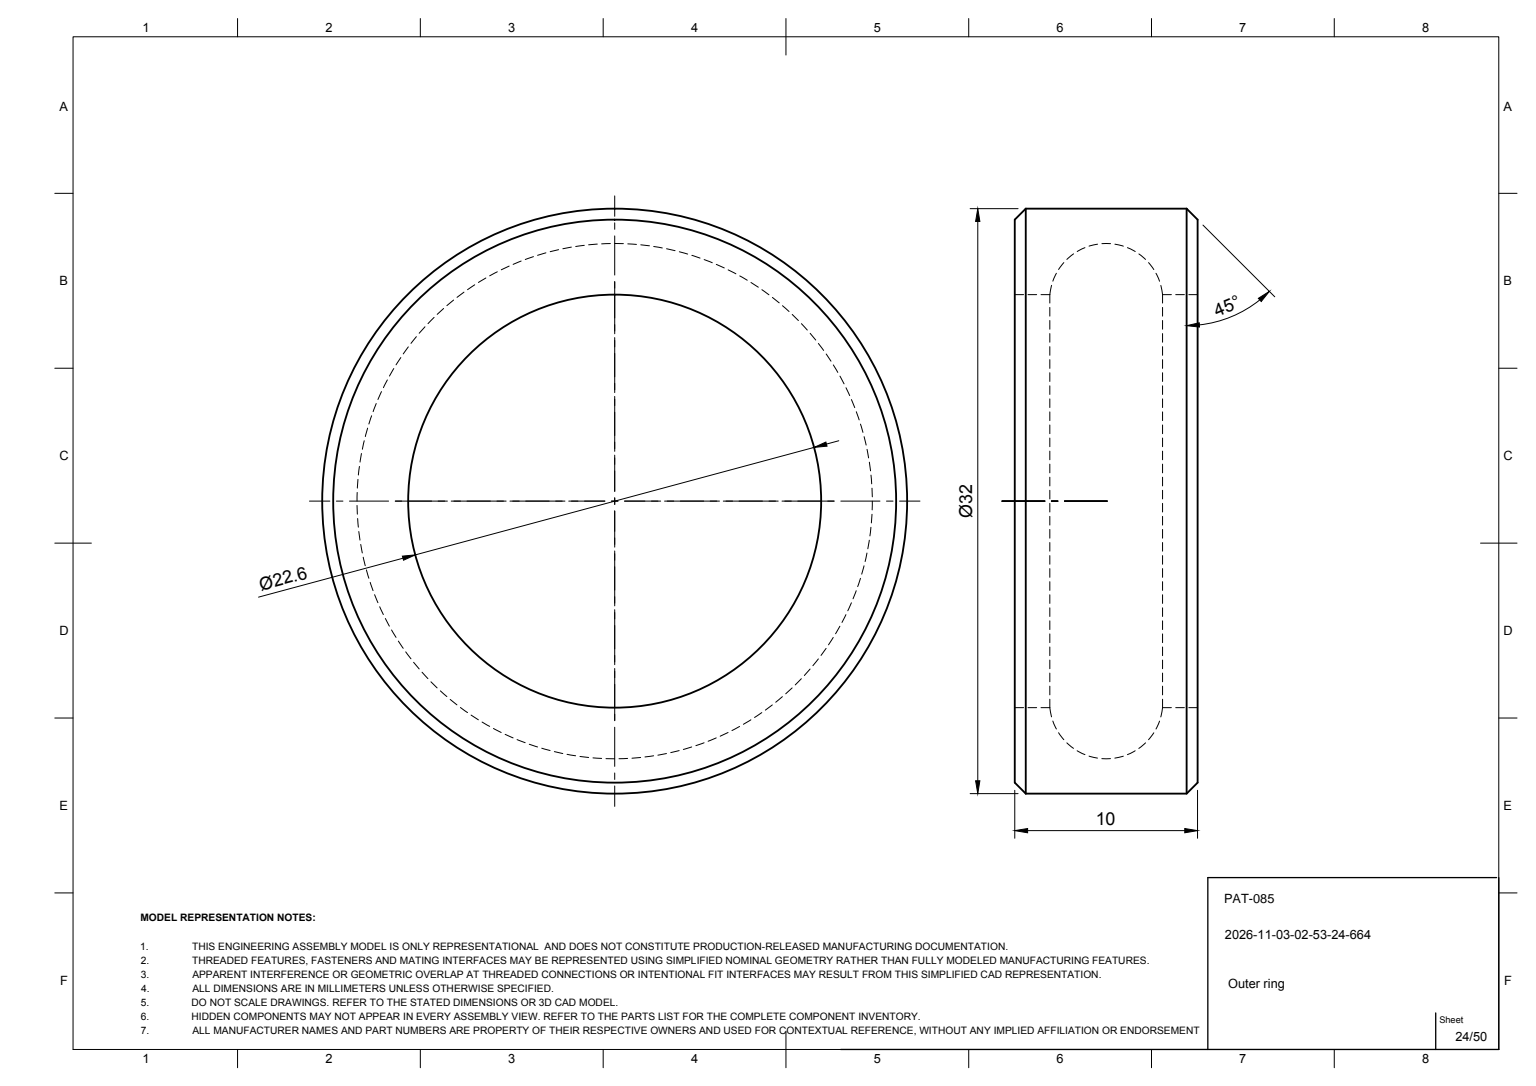
ISO-10303-21;
HEADER;
/* Generated by software containing ST-Developer
 * from STEP Tools, Inc. (www.steptools.com) 
 */

FILE_DESCRIPTION(
/* description */ ('Rack and pinion manual slide'),
/* implementation_level */ '2;1');

FILE_NAME(
/* name */ 'Outer ring.step',
/* time_stamp */ '2026-10-28T03:22:49-07:00',
/* author */ (''),
/* organization */ (''),
/* preprocessor_version */ 'ST-DEVELOPER v20.2',
/* originating_system */ 'Autodesk Translation Framework v15.17.0.0',
/* authorisation */ '');

FILE_SCHEMA (('AUTOMOTIVE_DESIGN { 1 0 10303 214 3 1 1 }'));
ENDSEC;

DATA;
#10=MECHANICAL_DESIGN_GEOMETRIC_PRESENTATION_REPRESENTATION('',(#752),#34851);
#604=TOROIDAL_SURFACE('',#14800,1.1,0.309556);
#622=CONICAL_SURFACE('',#14811,1.57,0.785398163397449);
#623=CONICAL_SURFACE('',#14815,1.57,0.785398163397449);
#660=SHAPE_REPRESENTATION_RELATIONSHIP('SRR','None',#35096,#706);
#706=ADVANCED_BREP_SHAPE_REPRESENTATION('',(#804),#34821);
#752=STYLED_ITEM('',(#35411),#804);
#804=MANIFOLD_SOLID_BREP('Body1',#13773);
#977=FACE_BOUND('',#2692,.T.);
#978=FACE_BOUND('',#2697,.T.);
#1220=PLANE('',#14808);
#1221=PLANE('',#14817);
#1806=FACE_OUTER_BOUND('',#2689,.T.);
#1807=FACE_OUTER_BOUND('',#2690,.T.);
#1808=FACE_OUTER_BOUND('',#2691,.T.);
#1809=FACE_OUTER_BOUND('',#2693,.T.);
#1810=FACE_OUTER_BOUND('',#2694,.T.);
#1811=FACE_OUTER_BOUND('',#2695,.T.);
#1812=FACE_OUTER_BOUND('',#2696,.T.);
#1813=FACE_OUTER_BOUND('',#2698,.T.);
#2689=EDGE_LOOP('',(#10522,#10523,#10524,#10525,#10526,#10527));
#2690=EDGE_LOOP('',(#10528,#10529,#10530,#10531,#10532));
#2691=EDGE_LOOP('',(#10533));
#2692=EDGE_LOOP('',(#10534));
#2693=EDGE_LOOP('',(#10535,#10536,#10537,#10538));
#2694=EDGE_LOOP('',(#10539,#10540,#10541,#10542));
#2695=EDGE_LOOP('',(#10543,#10544,#10545,#10546));
#2696=EDGE_LOOP('',(#10547));
#2697=EDGE_LOOP('',(#10548));
#2698=EDGE_LOOP('',(#10549,#10550,#10551,#10552,#10553));
#3680=LINE('',#20836,#4971);
#3681=LINE('',#20845,#4972);
#3682=LINE('',#20849,#4973);
#3683=LINE('',#20853,#4974);
#3684=LINE('',#20856,#4975);
#4971=VECTOR('',#17038,1.129765);
#4972=VECTOR('',#17049,1.57);
#4973=VECTOR('',#17054,1.6);
#4974=VECTOR('',#17059,1.57);
#4975=VECTOR('',#17064,1.129765);
#5992=CIRCLE('',#14801,1.129765);
#5993=CIRCLE('',#14802,1.129765);
#5994=CIRCLE('',#14803,0.309556);
#5995=CIRCLE('',#14804,1.129765);
#5996=CIRCLE('',#14805,1.129765);
#5997=CIRCLE('',#14807,1.129765);
#5998=CIRCLE('',#14809,1.54);
#5999=CIRCLE('',#14810,1.129765);
#6000=CIRCLE('',#14812,1.6);
#6001=CIRCLE('',#14814,1.6);
#6002=CIRCLE('',#14816,1.54);
#6651=VERTEX_POINT('',#20824);
#6652=VERTEX_POINT('',#20825);
#6653=VERTEX_POINT('',#20828);
#6654=VERTEX_POINT('',#20830);
#6655=VERTEX_POINT('',#20834);
#6656=VERTEX_POINT('',#20838);
#6657=VERTEX_POINT('',#20840);
#6658=VERTEX_POINT('',#20843);
#6659=VERTEX_POINT('',#20847);
#6660=VERTEX_POINT('',#20851);
#8073=EDGE_CURVE('',#6651,#6652,#5992,.T.);
#8074=EDGE_CURVE('',#6652,#6651,#5993,.T.);
#8075=EDGE_CURVE('',#6652,#6653,#5994,.T.);
#8076=EDGE_CURVE('',#6654,#6653,#5995,.T.);
#8077=EDGE_CURVE('',#6653,#6654,#5996,.T.);
#8078=EDGE_CURVE('',#6655,#6655,#5997,.T.);
#8079=EDGE_CURVE('',#6655,#6654,#3680,.T.);
#8080=EDGE_CURVE('',#6656,#6656,#5998,.T.);
#8081=EDGE_CURVE('',#6657,#6657,#5999,.T.);
#8082=EDGE_CURVE('',#6658,#6658,#6000,.T.);
#8083=EDGE_CURVE('',#6658,#6656,#3681,.T.);
#8084=EDGE_CURVE('',#6659,#6659,#6001,.T.);
#8085=EDGE_CURVE('',#6659,#6658,#3682,.T.);
#8086=EDGE_CURVE('',#6660,#6660,#6002,.T.);
#8087=EDGE_CURVE('',#6660,#6659,#3683,.T.);
#8088=EDGE_CURVE('',#6651,#6657,#3684,.T.);
#10522=ORIENTED_EDGE('',*,*,#8073,.F.);
#10523=ORIENTED_EDGE('',*,*,#8074,.F.);
#10524=ORIENTED_EDGE('',*,*,#8075,.T.);
#10525=ORIENTED_EDGE('',*,*,#8076,.F.);
#10526=ORIENTED_EDGE('',*,*,#8077,.F.);
#10527=ORIENTED_EDGE('',*,*,#8075,.F.);
#10528=ORIENTED_EDGE('',*,*,#8078,.T.);
#10529=ORIENTED_EDGE('',*,*,#8079,.T.);
#10530=ORIENTED_EDGE('',*,*,#8076,.T.);
#10531=ORIENTED_EDGE('',*,*,#8077,.T.);
#10532=ORIENTED_EDGE('',*,*,#8079,.F.);
#10533=ORIENTED_EDGE('',*,*,#8080,.F.);
#10534=ORIENTED_EDGE('',*,*,#8081,.T.);
#10535=ORIENTED_EDGE('',*,*,#8082,.F.);
#10536=ORIENTED_EDGE('',*,*,#8083,.T.);
#10537=ORIENTED_EDGE('',*,*,#8080,.T.);
#10538=ORIENTED_EDGE('',*,*,#8083,.F.);
#10539=ORIENTED_EDGE('',*,*,#8084,.F.);
#10540=ORIENTED_EDGE('',*,*,#8085,.T.);
#10541=ORIENTED_EDGE('',*,*,#8082,.T.);
#10542=ORIENTED_EDGE('',*,*,#8085,.F.);
#10543=ORIENTED_EDGE('',*,*,#8086,.F.);
#10544=ORIENTED_EDGE('',*,*,#8087,.T.);
#10545=ORIENTED_EDGE('',*,*,#8084,.T.);
#10546=ORIENTED_EDGE('',*,*,#8087,.F.);
#10547=ORIENTED_EDGE('',*,*,#8086,.T.);
#10548=ORIENTED_EDGE('',*,*,#8078,.F.);
#10549=ORIENTED_EDGE('',*,*,#8073,.T.);
#10550=ORIENTED_EDGE('',*,*,#8074,.T.);
#10551=ORIENTED_EDGE('',*,*,#8088,.T.);
#10552=ORIENTED_EDGE('',*,*,#8081,.F.);
#10553=ORIENTED_EDGE('',*,*,#8088,.F.);
#12931=CYLINDRICAL_SURFACE('',#14806,1.129765);
#12932=CYLINDRICAL_SURFACE('',#14813,1.6);
#12933=CYLINDRICAL_SURFACE('',#14818,1.129765);
#13284=ADVANCED_FACE('',(#1806),#604,.F.);
#13285=ADVANCED_FACE('',(#1807),#12931,.F.);
#13286=ADVANCED_FACE('',(#1808,#977),#1220,.T.);
#13287=ADVANCED_FACE('',(#1809),#622,.T.);
#13288=ADVANCED_FACE('',(#1810),#12932,.T.);
#13289=ADVANCED_FACE('',(#1811),#623,.T.);
#13290=ADVANCED_FACE('',(#1812,#978),#1221,.T.);
#13291=ADVANCED_FACE('',(#1813),#12933,.F.);
#13773=CLOSED_SHELL('',(#13284,#13285,#13286,#13287,#13288,#13289,#13290,
#13291));
#14799=AXIS2_PLACEMENT_3D('',#20822,#17020,#17021);
#14800=AXIS2_PLACEMENT_3D('',#20823,#17022,#17023);
#14801=AXIS2_PLACEMENT_3D('',#20826,#17024,#17025);
#14802=AXIS2_PLACEMENT_3D('',#20827,#17026,#17027);
#14803=AXIS2_PLACEMENT_3D('',#20829,#17028,#17029);
#14804=AXIS2_PLACEMENT_3D('',#20831,#17030,#17031);
#14805=AXIS2_PLACEMENT_3D('',#20832,#17032,#17033);
#14806=AXIS2_PLACEMENT_3D('',#20833,#17034,#17035);
#14807=AXIS2_PLACEMENT_3D('',#20835,#17036,#17037);
#14808=AXIS2_PLACEMENT_3D('',#20837,#17039,#17040);
#14809=AXIS2_PLACEMENT_3D('',#20839,#17041,#17042);
#14810=AXIS2_PLACEMENT_3D('',#20841,#17043,#17044);
#14811=AXIS2_PLACEMENT_3D('',#20842,#17045,#17046);
#14812=AXIS2_PLACEMENT_3D('',#20844,#17047,#17048);
#14813=AXIS2_PLACEMENT_3D('',#20846,#17050,#17051);
#14814=AXIS2_PLACEMENT_3D('',#20848,#17052,#17053);
#14815=AXIS2_PLACEMENT_3D('',#20850,#17055,#17056);
#14816=AXIS2_PLACEMENT_3D('',#20852,#17057,#17058);
#14817=AXIS2_PLACEMENT_3D('',#20854,#17060,#17061);
#14818=AXIS2_PLACEMENT_3D('',#20855,#17062,#17063);
#17020=DIRECTION('axis',(0.,0.,1.));
#17021=DIRECTION('refdir',(1.,0.,0.));
#17022=DIRECTION('center_axis',(0.,-1.,0.));
#17023=DIRECTION('ref_axis',(0.,0.,-1.));
#17024=DIRECTION('center_axis',(0.,-1.,0.));
#17025=DIRECTION('ref_axis',(1.,0.,0.));
#17026=DIRECTION('center_axis',(0.,-1.,0.));
#17027=DIRECTION('ref_axis',(1.,0.,0.));
#17028=DIRECTION('center_axis',(1.,0.,1.22464679914735E-16));
#17029=DIRECTION('ref_axis',(-1.22464679914735E-16,0.,1.));
#17030=DIRECTION('center_axis',(0.,1.,0.));
#17031=DIRECTION('ref_axis',(1.,0.,0.));
#17032=DIRECTION('center_axis',(0.,1.,0.));
#17033=DIRECTION('ref_axis',(1.,0.,0.));
#17034=DIRECTION('center_axis',(0.,-1.,0.));
#17035=DIRECTION('ref_axis',(1.,0.,0.));
#17036=DIRECTION('center_axis',(0.,-1.,0.));
#17037=DIRECTION('ref_axis',(1.,0.,0.));
#17038=DIRECTION('',(0.,1.,0.));
#17039=DIRECTION('center_axis',(0.,1.,0.));
#17040=DIRECTION('ref_axis',(0.,0.,1.));
#17041=DIRECTION('center_axis',(0.,-1.,0.));
#17042=DIRECTION('ref_axis',(1.,0.,0.));
#17043=DIRECTION('center_axis',(0.,-1.,0.));
#17044=DIRECTION('ref_axis',(1.,0.,0.));
#17045=DIRECTION('center_axis',(0.,-1.,0.));
#17046=DIRECTION('ref_axis',(1.,0.,0.));
#17047=DIRECTION('center_axis',(0.,-1.,0.));
#17048=DIRECTION('ref_axis',(1.,0.,0.));
#17049=DIRECTION('',(0.707106781186548,0.707106781186547,8.65956056235494E-17));
#17050=DIRECTION('center_axis',(0.,-1.,0.));
#17051=DIRECTION('ref_axis',(1.,0.,0.));
#17052=DIRECTION('center_axis',(0.,-1.,0.));
#17053=DIRECTION('ref_axis',(1.,0.,0.));
#17054=DIRECTION('',(0.,1.,0.));
#17055=DIRECTION('center_axis',(0.,1.,0.));
#17056=DIRECTION('ref_axis',(1.,0.,0.));
#17057=DIRECTION('center_axis',(0.,-1.,0.));
#17058=DIRECTION('ref_axis',(1.,0.,0.));
#17059=DIRECTION('',(-0.707106781186548,0.707106781186547,-8.65956056235494E-17));
#17060=DIRECTION('center_axis',(0.,-1.,0.));
#17061=DIRECTION('ref_axis',(0.,0.,-1.));
#17062=DIRECTION('center_axis',(0.,-1.,0.));
#17063=DIRECTION('ref_axis',(1.,0.,0.));
#17064=DIRECTION('',(0.,1.,0.));
#20822=CARTESIAN_POINT('',(0.,0.,0.));
#20823=CARTESIAN_POINT('Origin',(0.,0.,0.));
#20824=CARTESIAN_POINT('',(-1.129765,0.308121667383195,-1.38356309103871E-16));
#20825=CARTESIAN_POINT('',(-1.38356309103871E-16,0.308121667383195,1.129765));
#20826=CARTESIAN_POINT('Origin',(0.,0.308121667383195,0.));
#20827=CARTESIAN_POINT('Origin',(0.,0.308121667383195,0.));
#20828=CARTESIAN_POINT('',(-1.38356309103871E-16,-0.308121667383195,1.129765));
#20829=CARTESIAN_POINT('Origin',(-1.34711147906209E-16,0.,1.1));
#20830=CARTESIAN_POINT('',(-1.129765,-0.308121667383195,1.38356309103871E-16));
#20831=CARTESIAN_POINT('Origin',(0.,-0.308121667383195,0.));
#20832=CARTESIAN_POINT('Origin',(0.,-0.308121667383195,0.));
#20833=CARTESIAN_POINT('Origin',(0.,0.,0.));
#20834=CARTESIAN_POINT('',(-1.129765,-0.5,-1.38356309103871E-16));
#20835=CARTESIAN_POINT('Origin',(0.,-0.5,0.));
#20836=CARTESIAN_POINT('',(-1.129765,0.,-1.38356309103871E-16));
#20837=CARTESIAN_POINT('Origin',(1.54,0.5,0.));
#20838=CARTESIAN_POINT('',(-1.54,0.5,-1.88595607068692E-16));
#20839=CARTESIAN_POINT('Origin',(0.,0.5,0.));
#20840=CARTESIAN_POINT('',(-1.129765,0.5,-1.38356309103871E-16));
#20841=CARTESIAN_POINT('Origin',(0.,0.5,0.));
#20842=CARTESIAN_POINT('Origin',(0.,0.47,0.));
#20843=CARTESIAN_POINT('',(-1.6,0.44,-1.95943487863577E-16));
#20844=CARTESIAN_POINT('Origin',(0.,0.44,0.));
#20845=CARTESIAN_POINT('',(-1.57,0.47,-1.92269547466134E-16));
#20846=CARTESIAN_POINT('Origin',(0.,0.,0.));
#20847=CARTESIAN_POINT('',(-1.6,-0.44,-1.95943487863577E-16));
#20848=CARTESIAN_POINT('Origin',(0.,-0.44,0.));
#20849=CARTESIAN_POINT('',(-1.6,0.,-1.95943487863577E-16));
#20850=CARTESIAN_POINT('Origin',(0.,-0.47,0.));
#20851=CARTESIAN_POINT('',(-1.54,-0.5,-1.88595607068692E-16));
#20852=CARTESIAN_POINT('Origin',(0.,-0.5,0.));
#20853=CARTESIAN_POINT('',(-1.57,-0.47,-1.92269547466134E-16));
#20854=CARTESIAN_POINT('Origin',(1.129765,-0.5,0.));
#20855=CARTESIAN_POINT('Origin',(0.,0.,0.));
#20856=CARTESIAN_POINT('',(-1.129765,0.,-1.38356309103871E-16));
#34767=UNCERTAINTY_MEASURE_WITH_UNIT(LENGTH_MEASURE(0.001),#34852,
'DISTANCE_ACCURACY_VALUE',
'Maximum model space distance between geometric entities at asserted c
onnectivities');
#34797=UNCERTAINTY_MEASURE_WITH_UNIT(LENGTH_MEASURE(0.001),#34852,
'DISTANCE_ACCURACY_VALUE',
'Maximum model space distance between geometric entities at asserted c
onnectivities');
#34821=(
GEOMETRIC_REPRESENTATION_CONTEXT(3)
GLOBAL_UNCERTAINTY_ASSIGNED_CONTEXT((#34767))
GLOBAL_UNIT_ASSIGNED_CONTEXT((#34852,#34854,#34855))
REPRESENTATION_CONTEXT('','3D')
);
#34851=(
GEOMETRIC_REPRESENTATION_CONTEXT(3)
GLOBAL_UNCERTAINTY_ASSIGNED_CONTEXT((#34797))
GLOBAL_UNIT_ASSIGNED_CONTEXT((#34852,#34854,#34855))
REPRESENTATION_CONTEXT('','3D')
);
#34852=(
LENGTH_UNIT()
NAMED_UNIT(*)
SI_UNIT(.CENTI.,.METRE.)
);
#34854=(
NAMED_UNIT(*)
PLANE_ANGLE_UNIT()
SI_UNIT($,.RADIAN.)
);
#34855=(
NAMED_UNIT(*)
SI_UNIT($,.STERADIAN.)
SOLID_ANGLE_UNIT()
);
#34879=SHAPE_DEFINITION_REPRESENTATION(#34932,#35096);
#34932=PRODUCT_DEFINITION_SHAPE('',$,#35150);
#35096=SHAPE_REPRESENTATION('',(#14799),#34821);
#35126=PRODUCT_DEFINITION_CONTEXT('part definition',#35287,'design');
#35150=PRODUCT_DEFINITION('Outer ring','Outer ring',#35203,#35126);
#35203=PRODUCT_DEFINITION_FORMATION('',$,#35312);
#35287=APPLICATION_CONTEXT(
'Core Data for Automotive Mechanical Design Process');
#35288=PRODUCT_CONTEXT('part definition',#35287,'mechanical');
#35312=PRODUCT('Outer ring','Outer ring','Outer ring',(#35288));
#35405=COLOUR_RGB('Grey',0.48,0.52,0.57);
#35406=FILL_AREA_STYLE_COLOUR('',#35405);
#35407=FILL_AREA_STYLE('',(#35406));
#35408=SURFACE_STYLE_FILL_AREA(#35407);
#35409=SURFACE_SIDE_STYLE('',(#35408));
#35410=SURFACE_STYLE_USAGE(.BOTH.,#35409);
#35411=PRESENTATION_STYLE_ASSIGNMENT((#35410));
ENDSEC;
END-ISO-10303-21;
